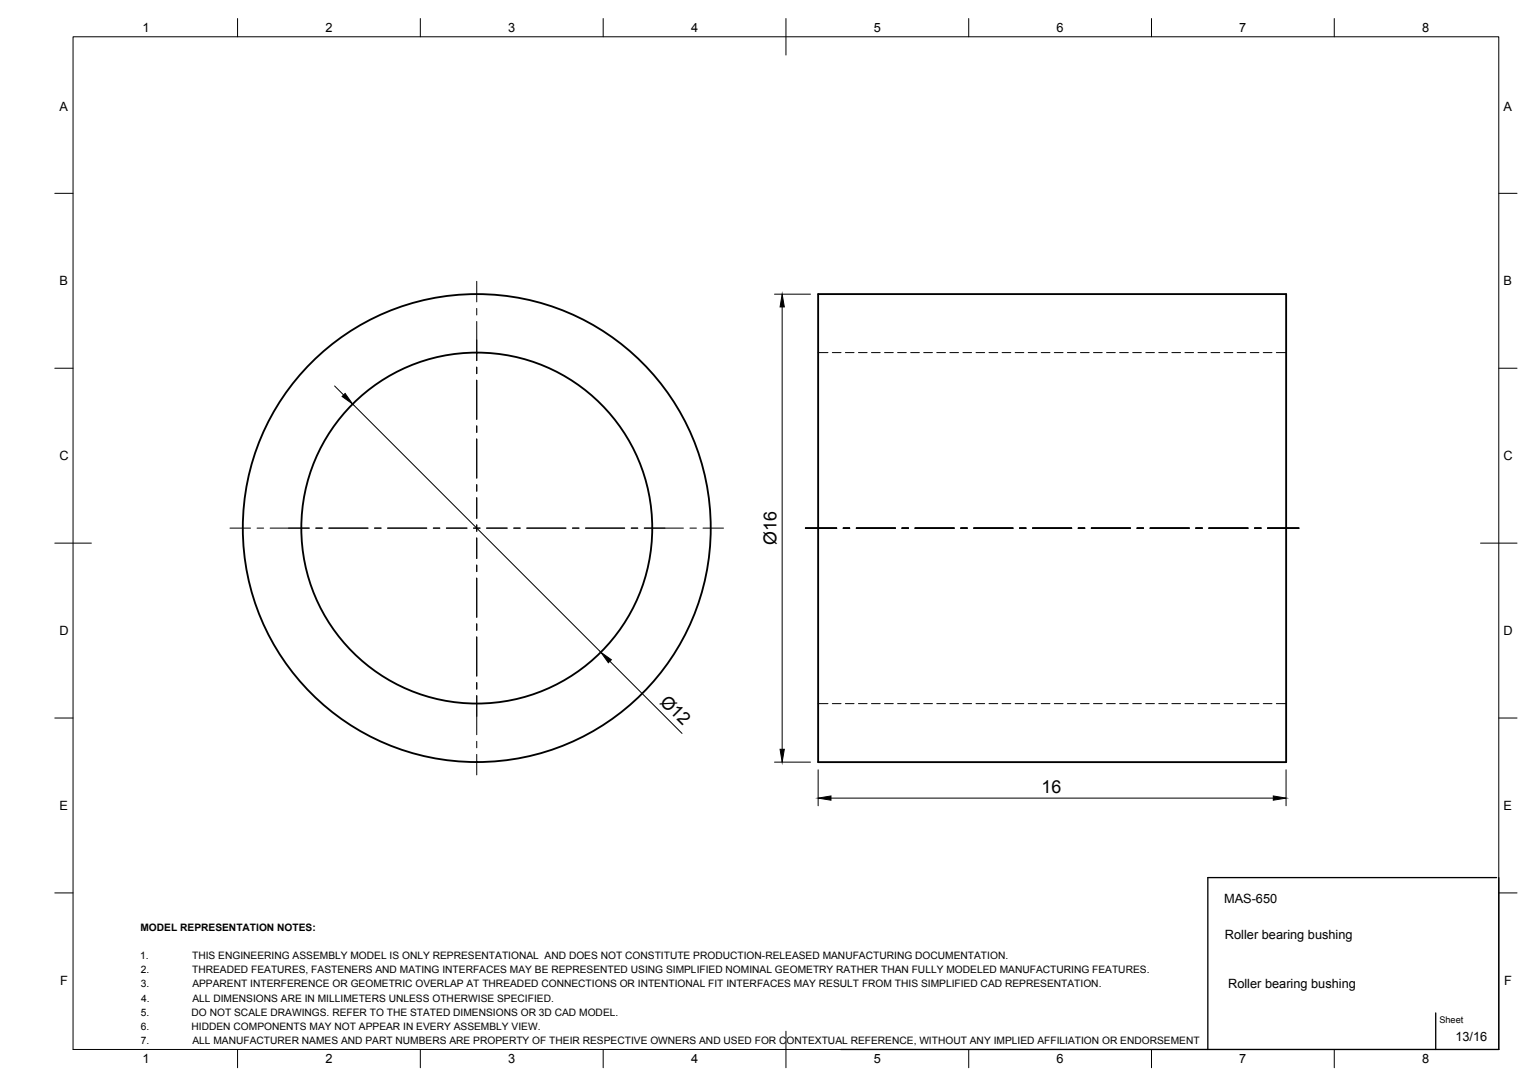
ISO-10303-21;
HEADER;
/* Generated by software containing ST-Developer
 * from STEP Tools, Inc. (www.steptools.com) 
 */

FILE_DESCRIPTION(
/* description */ ('Independent manual traversing gantry with native reusable aluminum pr
ofiles,180mm captured carriage travel, four bronze-bushed rollers, lin
ked ideal rolling motion, bonded acetal lateral guides, positive welde
d end stops and fully retained axle stacks. Editable native profile cu
t lengths220/400mm. Tool attachments viaM6 bridge-plate taps; mounted 
tool outside assembly. Welds, anchors, adhesives, fits, traction, load
/speed/structural/life ratings unassigned.'),
/* implementation_level */ '2;1');

FILE_NAME(
/* name */ 'Roller bearing bushing.step',
/* time_stamp */ '2026-11-09T20:04:38-08:00',
/* author */ (''),
/* organization */ (''),
/* preprocessor_version */ 'ST-DEVELOPER v20.2',
/* originating_system */ 'Autodesk Translation Framework v15.17.0.0',
/* authorisation */ '');

FILE_SCHEMA (('AUTOMOTIVE_DESIGN { 1 0 10303 214 3 1 1 }'));
ENDSEC;

DATA;
#10=MECHANICAL_DESIGN_GEOMETRIC_PRESENTATION_REPRESENTATION('',(#481),#13231);
#449=SHAPE_REPRESENTATION_RELATIONSHIP('SRR','None',#13338,#465);
#465=ADVANCED_BREP_SHAPE_REPRESENTATION('',(#497),#13225);
#481=STYLED_ITEM('',(#13426),#497);
#497=MANIFOLD_SOLID_BREP('Body1',#4161);
#541=FACE_BOUND('',#1085,.T.);
#542=FACE_BOUND('',#1087,.T.);
#616=PLANE('',#4620);
#617=PLANE('',#4621);
#823=FACE_OUTER_BOUND('',#1082,.T.);
#824=FACE_OUTER_BOUND('',#1083,.T.);
#825=FACE_OUTER_BOUND('',#1084,.T.);
#826=FACE_OUTER_BOUND('',#1086,.T.);
#1082=EDGE_LOOP('',(#3702,#3703,#3704,#3705));
#1083=EDGE_LOOP('',(#3706,#3707,#3708,#3709));
#1084=EDGE_LOOP('',(#3710));
#1085=EDGE_LOOP('',(#3711));
#1086=EDGE_LOOP('',(#3712));
#1087=EDGE_LOOP('',(#3713));
#1366=LINE('',#13027,#1628);
#1367=LINE('',#13033,#1629);
#1628=VECTOR('',#5521,6.);
#1629=VECTOR('',#5528,8.);
#1724=CIRCLE('',#4615,6.);
#1725=CIRCLE('',#4616,6.);
#1726=CIRCLE('',#4618,8.);
#1727=CIRCLE('',#4619,8.);
#2092=VERTEX_POINT('',#13024);
#2093=VERTEX_POINT('',#13026);
#2094=VERTEX_POINT('',#13030);
#2095=VERTEX_POINT('',#13032);
#2634=EDGE_CURVE('',#2092,#2092,#1724,.T.);
#2635=EDGE_CURVE('',#2092,#2093,#1366,.T.);
#2636=EDGE_CURVE('',#2093,#2093,#1725,.T.);
#2637=EDGE_CURVE('',#2094,#2094,#1726,.T.);
#2638=EDGE_CURVE('',#2094,#2095,#1367,.T.);
#2639=EDGE_CURVE('',#2095,#2095,#1727,.T.);
#3702=ORIENTED_EDGE('',*,*,#2634,.F.);
#3703=ORIENTED_EDGE('',*,*,#2635,.T.);
#3704=ORIENTED_EDGE('',*,*,#2636,.T.);
#3705=ORIENTED_EDGE('',*,*,#2635,.F.);
#3706=ORIENTED_EDGE('',*,*,#2637,.F.);
#3707=ORIENTED_EDGE('',*,*,#2638,.T.);
#3708=ORIENTED_EDGE('',*,*,#2639,.T.);
#3709=ORIENTED_EDGE('',*,*,#2638,.F.);
#3710=ORIENTED_EDGE('',*,*,#2637,.T.);
#3711=ORIENTED_EDGE('',*,*,#2634,.T.);
#3712=ORIENTED_EDGE('',*,*,#2639,.F.);
#3713=ORIENTED_EDGE('',*,*,#2636,.F.);
#3916=CYLINDRICAL_SURFACE('',#4614,6.);
#3917=CYLINDRICAL_SURFACE('',#4617,8.);
#4120=ADVANCED_FACE('',(#823),#3916,.F.);
#4121=ADVANCED_FACE('',(#824),#3917,.T.);
#4122=ADVANCED_FACE('',(#825,#541),#616,.T.);
#4123=ADVANCED_FACE('',(#826,#542),#617,.F.);
#4161=CLOSED_SHELL('',(#4120,#4121,#4122,#4123));
#4613=AXIS2_PLACEMENT_3D('',#13022,#5515,#5516);
#4614=AXIS2_PLACEMENT_3D('',#13023,#5517,#5518);
#4615=AXIS2_PLACEMENT_3D('',#13025,#5519,#5520);
#4616=AXIS2_PLACEMENT_3D('',#13028,#5522,#5523);
#4617=AXIS2_PLACEMENT_3D('',#13029,#5524,#5525);
#4618=AXIS2_PLACEMENT_3D('',#13031,#5526,#5527);
#4619=AXIS2_PLACEMENT_3D('',#13034,#5529,#5530);
#4620=AXIS2_PLACEMENT_3D('',#13035,#5531,#5532);
#4621=AXIS2_PLACEMENT_3D('',#13036,#5533,#5534);
#5515=DIRECTION('axis',(0.,0.,1.));
#5516=DIRECTION('refdir',(1.,0.,0.));
#5517=DIRECTION('center_axis',(0.,0.,1.));
#5518=DIRECTION('ref_axis',(1.,0.,0.));
#5519=DIRECTION('center_axis',(0.,0.,-1.));
#5520=DIRECTION('ref_axis',(1.,0.,0.));
#5521=DIRECTION('',(0.,0.,-1.));
#5522=DIRECTION('center_axis',(0.,0.,-1.));
#5523=DIRECTION('ref_axis',(1.,0.,0.));
#5524=DIRECTION('center_axis',(0.,0.,1.));
#5525=DIRECTION('ref_axis',(1.,0.,0.));
#5526=DIRECTION('center_axis',(0.,0.,1.));
#5527=DIRECTION('ref_axis',(1.,0.,0.));
#5528=DIRECTION('',(0.,0.,-1.));
#5529=DIRECTION('center_axis',(0.,0.,1.));
#5530=DIRECTION('ref_axis',(1.,0.,0.));
#5531=DIRECTION('center_axis',(0.,0.,1.));
#5532=DIRECTION('ref_axis',(1.,0.,0.));
#5533=DIRECTION('center_axis',(0.,0.,1.));
#5534=DIRECTION('ref_axis',(1.,0.,0.));
#13022=CARTESIAN_POINT('',(0.,0.,0.));
#13023=CARTESIAN_POINT('Origin',(0.,0.,0.));
#13024=CARTESIAN_POINT('',(-6.,-7.34788079488412E-16,16.));
#13025=CARTESIAN_POINT('Origin',(0.,0.,16.));
#13026=CARTESIAN_POINT('',(-6.,-7.34788079488412E-16,0.));
#13027=CARTESIAN_POINT('',(-6.,-7.34788079488412E-16,0.));
#13028=CARTESIAN_POINT('Origin',(0.,0.,0.));
#13029=CARTESIAN_POINT('Origin',(0.,0.,0.));
#13030=CARTESIAN_POINT('',(-8.,-9.79717439317883E-16,16.));
#13031=CARTESIAN_POINT('Origin',(0.,0.,16.));
#13032=CARTESIAN_POINT('',(-8.,-9.79717439317883E-16,0.));
#13033=CARTESIAN_POINT('',(-8.,-9.79717439317883E-16,0.));
#13034=CARTESIAN_POINT('Origin',(0.,0.,0.));
#13035=CARTESIAN_POINT('Origin',(0.,0.,16.));
#13036=CARTESIAN_POINT('Origin',(0.,0.,0.));
#13207=UNCERTAINTY_MEASURE_WITH_UNIT(LENGTH_MEASURE(0.01),#13232,
'DISTANCE_ACCURACY_VALUE',
'Maximum model space distance between geometric entities at asserted c
onnectivities');
#13213=UNCERTAINTY_MEASURE_WITH_UNIT(LENGTH_MEASURE(0.01),#13232,
'DISTANCE_ACCURACY_VALUE',
'Maximum model space distance between geometric entities at asserted c
onnectivities');
#13225=(
GEOMETRIC_REPRESENTATION_CONTEXT(3)
GLOBAL_UNCERTAINTY_ASSIGNED_CONTEXT((#13207))
GLOBAL_UNIT_ASSIGNED_CONTEXT((#13232,#13234,#13235))
REPRESENTATION_CONTEXT('','3D')
);
#13231=(
GEOMETRIC_REPRESENTATION_CONTEXT(3)
GLOBAL_UNCERTAINTY_ASSIGNED_CONTEXT((#13213))
GLOBAL_UNIT_ASSIGNED_CONTEXT((#13232,#13234,#13235))
REPRESENTATION_CONTEXT('','3D')
);
#13232=(
LENGTH_UNIT()
NAMED_UNIT(*)
SI_UNIT(.MILLI.,.METRE.)
);
#13234=(
NAMED_UNIT(*)
PLANE_ANGLE_UNIT()
SI_UNIT($,.RADIAN.)
);
#13235=(
NAMED_UNIT(*)
SI_UNIT($,.STERADIAN.)
SOLID_ANGLE_UNIT()
);
#13247=SHAPE_DEFINITION_REPRESENTATION(#13264,#13338);
#13264=PRODUCT_DEFINITION_SHAPE('',$,#13356);
#13338=SHAPE_REPRESENTATION('',(#4613),#13225);
#13344=PRODUCT_DEFINITION_CONTEXT('part definition',#13397,'design');
#13356=PRODUCT_DEFINITION('Roller bearing bushing',
'Roller bearing bushing',#13373,#13344);
#13373=PRODUCT_DEFINITION_FORMATION('',$,#13410);
#13397=APPLICATION_CONTEXT(
'Core Data for Automotive Mechanical Design Process');
#13398=PRODUCT_CONTEXT('part definition',#13397,'mechanical');
#13410=PRODUCT('Roller bearing bushing','Roller bearing bushing',$,(#13398));
#13426=PRESENTATION_STYLE_ASSIGNMENT((#13440));
#13440=SURFACE_STYLE_USAGE(.BOTH.,#13454);
#13454=SURFACE_SIDE_STYLE('',(#13468));
#13468=SURFACE_STYLE_FILL_AREA(#13482);
#13482=FILL_AREA_STYLE('Bearing gray',(#13496));
#13496=FILL_AREA_STYLE_COLOUR('Bearing gray',#13510);
#13510=COLOUR_RGB('Bearing gray',0.725490196078431,0.752941176470588,0.792156862745098);
ENDSEC;
END-ISO-10303-21;
